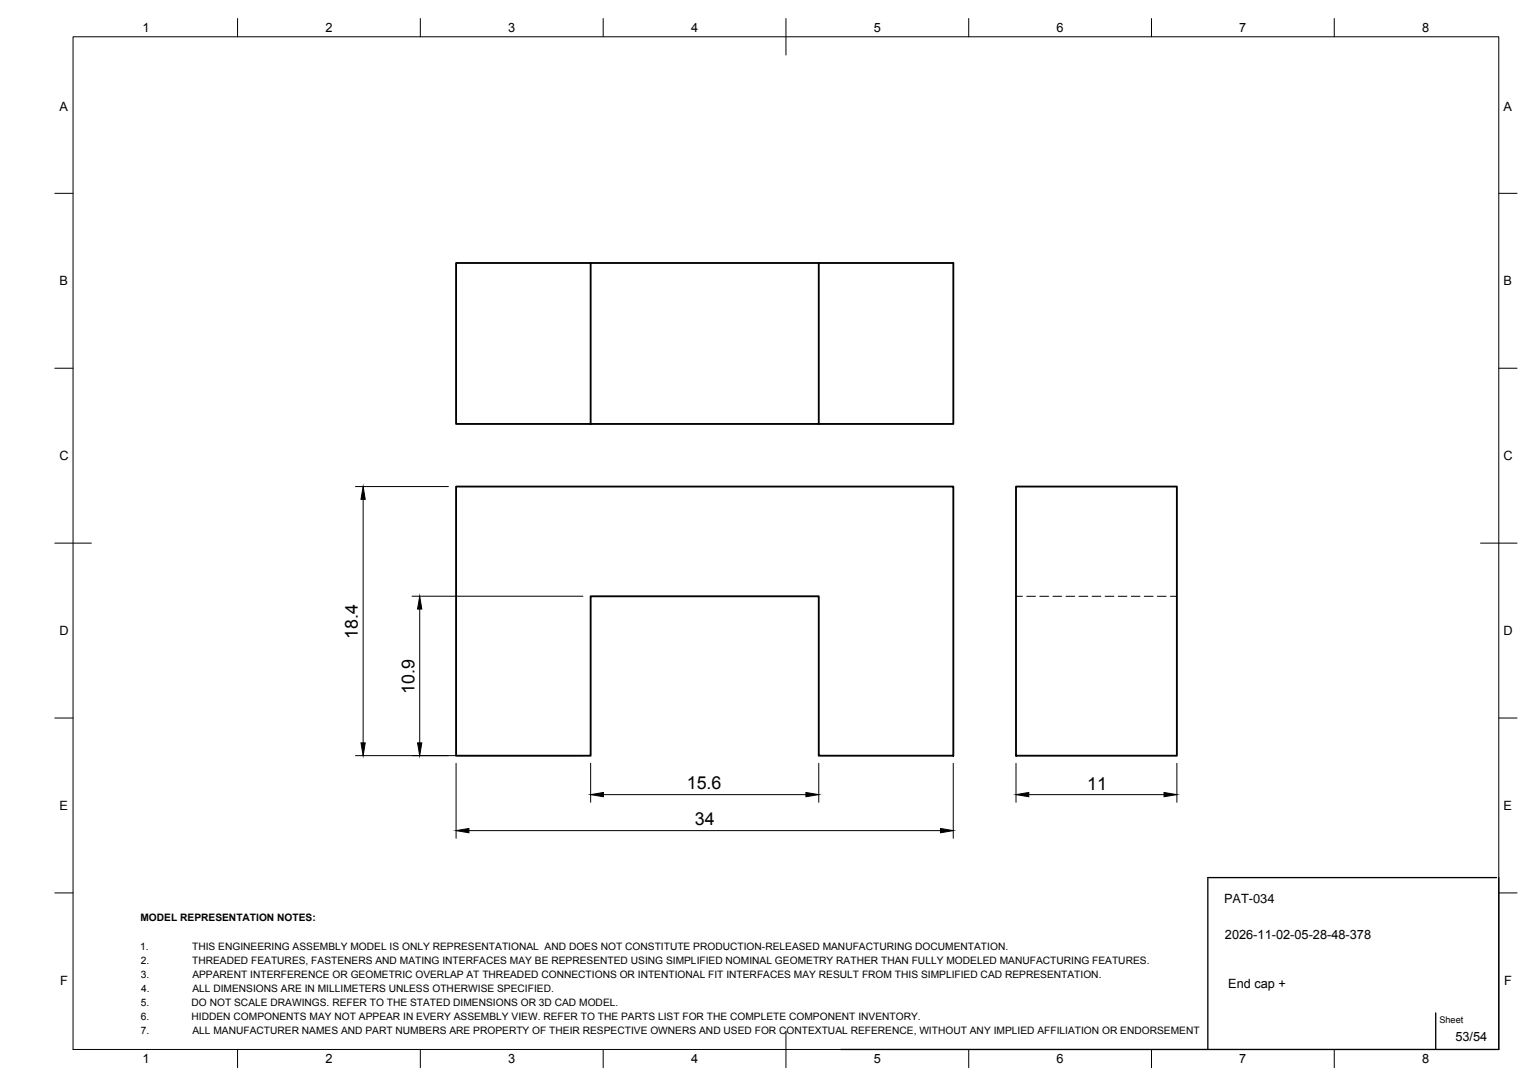
ISO-10303-21;
HEADER;
/* Generated by software containing ST-Developer
 * from STEP Tools, Inc. (www.steptools.com) 
 */

FILE_DESCRIPTION(
/* description */ ('Fatigue rig crank-slider'),
/* implementation_level */ '2;1');

FILE_NAME(
/* name */ 'End cap +.step',
/* time_stamp */ '2026-10-28T03:24:50-07:00',
/* author */ (''),
/* organization */ (''),
/* preprocessor_version */ 'ST-DEVELOPER v20.2',
/* originating_system */ 'Autodesk Translation Framework v15.17.0.0',
/* authorisation */ '');

FILE_SCHEMA (('AUTOMOTIVE_DESIGN { 1 0 10303 214 3 1 1 }'));
ENDSEC;

DATA;
#10=MECHANICAL_DESIGN_GEOMETRIC_PRESENTATION_REPRESENTATION('',(#640),#16911);
#531=SHAPE_REPRESENTATION_RELATIONSHIP('SRR','None',#17176,#581);
#581=ADVANCED_BREP_SHAPE_REPRESENTATION('',(#697),#16905);
#640=STYLED_ITEM('',(#17480),#697);
#697=MANIFOLD_SOLID_BREP('Body1',#8933);
#1162=PLANE('',#10382);
#1163=PLANE('',#10383);
#1164=PLANE('',#10384);
#1165=PLANE('',#10385);
#1166=PLANE('',#10386);
#1167=PLANE('',#10387);
#1168=PLANE('',#10388);
#1169=PLANE('',#10389);
#1170=PLANE('',#10390);
#1171=PLANE('',#10391);
#1666=FACE_OUTER_BOUND('',#2381,.T.);
#1667=FACE_OUTER_BOUND('',#2382,.T.);
#1668=FACE_OUTER_BOUND('',#2383,.T.);
#1669=FACE_OUTER_BOUND('',#2384,.T.);
#1670=FACE_OUTER_BOUND('',#2385,.T.);
#1671=FACE_OUTER_BOUND('',#2386,.T.);
#1672=FACE_OUTER_BOUND('',#2387,.T.);
#1673=FACE_OUTER_BOUND('',#2388,.T.);
#1674=FACE_OUTER_BOUND('',#2389,.T.);
#1675=FACE_OUTER_BOUND('',#2390,.T.);
#2381=EDGE_LOOP('',(#7900,#7901,#7902,#7903));
#2382=EDGE_LOOP('',(#7904,#7905,#7906,#7907));
#2383=EDGE_LOOP('',(#7908,#7909,#7910,#7911));
#2384=EDGE_LOOP('',(#7912,#7913,#7914,#7915));
#2385=EDGE_LOOP('',(#7916,#7917,#7918,#7919));
#2386=EDGE_LOOP('',(#7920,#7921,#7922,#7923));
#2387=EDGE_LOOP('',(#7924,#7925,#7926,#7927));
#2388=EDGE_LOOP('',(#7928,#7929,#7930,#7931));
#2389=EDGE_LOOP('',(#7932,#7933,#7934,#7935,#7936,#7937,#7938,#7939));
#2390=EDGE_LOOP('',(#7940,#7941,#7942,#7943,#7944,#7945,#7946,#7947));
#2985=LINE('',#16397,#3631);
#2986=LINE('',#16399,#3632);
#2987=LINE('',#16401,#3633);
#2988=LINE('',#16402,#3634);
#2989=LINE('',#16405,#3635);
#2990=LINE('',#16407,#3636);
#2991=LINE('',#16408,#3637);
#2992=LINE('',#16411,#3638);
#2993=LINE('',#16413,#3639);
#2994=LINE('',#16414,#3640);
#2995=LINE('',#16417,#3641);
#2996=LINE('',#16419,#3642);
#2997=LINE('',#16420,#3643);
#2998=LINE('',#16423,#3644);
#2999=LINE('',#16425,#3645);
#3000=LINE('',#16426,#3646);
#3001=LINE('',#16429,#3647);
#3002=LINE('',#16431,#3648);
#3003=LINE('',#16432,#3649);
#3004=LINE('',#16435,#3650);
#3005=LINE('',#16437,#3651);
#3006=LINE('',#16438,#3652);
#3007=LINE('',#16440,#3653);
#3008=LINE('',#16441,#3654);
#3631=VECTOR('',#12871,1.);
#3632=VECTOR('',#12872,1.);
#3633=VECTOR('',#12873,1.);
#3634=VECTOR('',#12874,1.);
#3635=VECTOR('',#12877,1.);
#3636=VECTOR('',#12878,1.);
#3637=VECTOR('',#12879,1.);
#3638=VECTOR('',#12882,1.);
#3639=VECTOR('',#12883,1.);
#3640=VECTOR('',#12884,1.);
#3641=VECTOR('',#12887,1.);
#3642=VECTOR('',#12888,1.);
#3643=VECTOR('',#12889,1.);
#3644=VECTOR('',#12892,1.);
#3645=VECTOR('',#12893,1.);
#3646=VECTOR('',#12894,1.);
#3647=VECTOR('',#12897,1.);
#3648=VECTOR('',#12898,1.);
#3649=VECTOR('',#12899,1.);
#3650=VECTOR('',#12902,1.);
#3651=VECTOR('',#12903,1.);
#3652=VECTOR('',#12904,1.);
#3653=VECTOR('',#12907,1.);
#3654=VECTOR('',#12908,1.);
#4801=VERTEX_POINT('',#16395);
#4802=VERTEX_POINT('',#16396);
#4803=VERTEX_POINT('',#16398);
#4804=VERTEX_POINT('',#16400);
#4805=VERTEX_POINT('',#16404);
#4806=VERTEX_POINT('',#16406);
#4807=VERTEX_POINT('',#16410);
#4808=VERTEX_POINT('',#16412);
#4809=VERTEX_POINT('',#16416);
#4810=VERTEX_POINT('',#16418);
#4811=VERTEX_POINT('',#16422);
#4812=VERTEX_POINT('',#16424);
#4813=VERTEX_POINT('',#16428);
#4814=VERTEX_POINT('',#16430);
#4815=VERTEX_POINT('',#16434);
#4816=VERTEX_POINT('',#16436);
#5848=EDGE_CURVE('',#4801,#4802,#2985,.T.);
#5849=EDGE_CURVE('',#4802,#4803,#2986,.T.);
#5850=EDGE_CURVE('',#4804,#4803,#2987,.T.);
#5851=EDGE_CURVE('',#4801,#4804,#2988,.T.);
#5852=EDGE_CURVE('',#4805,#4801,#2989,.T.);
#5853=EDGE_CURVE('',#4806,#4804,#2990,.T.);
#5854=EDGE_CURVE('',#4805,#4806,#2991,.T.);
#5855=EDGE_CURVE('',#4807,#4805,#2992,.T.);
#5856=EDGE_CURVE('',#4808,#4806,#2993,.T.);
#5857=EDGE_CURVE('',#4807,#4808,#2994,.T.);
#5858=EDGE_CURVE('',#4809,#4807,#2995,.T.);
#5859=EDGE_CURVE('',#4810,#4808,#2996,.T.);
#5860=EDGE_CURVE('',#4809,#4810,#2997,.T.);
#5861=EDGE_CURVE('',#4811,#4809,#2998,.T.);
#5862=EDGE_CURVE('',#4812,#4810,#2999,.T.);
#5863=EDGE_CURVE('',#4811,#4812,#3000,.T.);
#5864=EDGE_CURVE('',#4813,#4811,#3001,.T.);
#5865=EDGE_CURVE('',#4814,#4812,#3002,.T.);
#5866=EDGE_CURVE('',#4813,#4814,#3003,.T.);
#5867=EDGE_CURVE('',#4815,#4813,#3004,.T.);
#5868=EDGE_CURVE('',#4816,#4814,#3005,.T.);
#5869=EDGE_CURVE('',#4815,#4816,#3006,.T.);
#5870=EDGE_CURVE('',#4802,#4815,#3007,.T.);
#5871=EDGE_CURVE('',#4803,#4816,#3008,.T.);
#7900=ORIENTED_EDGE('',*,*,#5848,.T.);
#7901=ORIENTED_EDGE('',*,*,#5849,.T.);
#7902=ORIENTED_EDGE('',*,*,#5850,.F.);
#7903=ORIENTED_EDGE('',*,*,#5851,.F.);
#7904=ORIENTED_EDGE('',*,*,#5852,.T.);
#7905=ORIENTED_EDGE('',*,*,#5851,.T.);
#7906=ORIENTED_EDGE('',*,*,#5853,.F.);
#7907=ORIENTED_EDGE('',*,*,#5854,.F.);
#7908=ORIENTED_EDGE('',*,*,#5855,.T.);
#7909=ORIENTED_EDGE('',*,*,#5854,.T.);
#7910=ORIENTED_EDGE('',*,*,#5856,.F.);
#7911=ORIENTED_EDGE('',*,*,#5857,.F.);
#7912=ORIENTED_EDGE('',*,*,#5858,.T.);
#7913=ORIENTED_EDGE('',*,*,#5857,.T.);
#7914=ORIENTED_EDGE('',*,*,#5859,.F.);
#7915=ORIENTED_EDGE('',*,*,#5860,.F.);
#7916=ORIENTED_EDGE('',*,*,#5861,.T.);
#7917=ORIENTED_EDGE('',*,*,#5860,.T.);
#7918=ORIENTED_EDGE('',*,*,#5862,.F.);
#7919=ORIENTED_EDGE('',*,*,#5863,.F.);
#7920=ORIENTED_EDGE('',*,*,#5864,.T.);
#7921=ORIENTED_EDGE('',*,*,#5863,.T.);
#7922=ORIENTED_EDGE('',*,*,#5865,.F.);
#7923=ORIENTED_EDGE('',*,*,#5866,.F.);
#7924=ORIENTED_EDGE('',*,*,#5867,.T.);
#7925=ORIENTED_EDGE('',*,*,#5866,.T.);
#7926=ORIENTED_EDGE('',*,*,#5868,.F.);
#7927=ORIENTED_EDGE('',*,*,#5869,.F.);
#7928=ORIENTED_EDGE('',*,*,#5870,.T.);
#7929=ORIENTED_EDGE('',*,*,#5869,.T.);
#7930=ORIENTED_EDGE('',*,*,#5871,.F.);
#7931=ORIENTED_EDGE('',*,*,#5849,.F.);
#7932=ORIENTED_EDGE('',*,*,#5871,.T.);
#7933=ORIENTED_EDGE('',*,*,#5868,.T.);
#7934=ORIENTED_EDGE('',*,*,#5865,.T.);
#7935=ORIENTED_EDGE('',*,*,#5862,.T.);
#7936=ORIENTED_EDGE('',*,*,#5859,.T.);
#7937=ORIENTED_EDGE('',*,*,#5856,.T.);
#7938=ORIENTED_EDGE('',*,*,#5853,.T.);
#7939=ORIENTED_EDGE('',*,*,#5850,.T.);
#7940=ORIENTED_EDGE('',*,*,#5870,.F.);
#7941=ORIENTED_EDGE('',*,*,#5848,.F.);
#7942=ORIENTED_EDGE('',*,*,#5852,.F.);
#7943=ORIENTED_EDGE('',*,*,#5855,.F.);
#7944=ORIENTED_EDGE('',*,*,#5858,.F.);
#7945=ORIENTED_EDGE('',*,*,#5861,.F.);
#7946=ORIENTED_EDGE('',*,*,#5864,.F.);
#7947=ORIENTED_EDGE('',*,*,#5867,.F.);
#8804=ADVANCED_FACE('',(#1666),#1162,.T.);
#8805=ADVANCED_FACE('',(#1667),#1163,.T.);
#8806=ADVANCED_FACE('',(#1668),#1164,.T.);
#8807=ADVANCED_FACE('',(#1669),#1165,.T.);
#8808=ADVANCED_FACE('',(#1670),#1166,.T.);
#8809=ADVANCED_FACE('',(#1671),#1167,.T.);
#8810=ADVANCED_FACE('',(#1672),#1168,.T.);
#8811=ADVANCED_FACE('',(#1673),#1169,.T.);
#8812=ADVANCED_FACE('',(#1674),#1170,.T.);
#8813=ADVANCED_FACE('',(#1675),#1171,.F.);
#8933=CLOSED_SHELL('',(#8804,#8805,#8806,#8807,#8808,#8809,#8810,#8811,
#8812,#8813));
#10381=AXIS2_PLACEMENT_3D('',#16393,#12867,#12868);
#10382=AXIS2_PLACEMENT_3D('',#16394,#12869,#12870);
#10383=AXIS2_PLACEMENT_3D('',#16403,#12875,#12876);
#10384=AXIS2_PLACEMENT_3D('',#16409,#12880,#12881);
#10385=AXIS2_PLACEMENT_3D('',#16415,#12885,#12886);
#10386=AXIS2_PLACEMENT_3D('',#16421,#12890,#12891);
#10387=AXIS2_PLACEMENT_3D('',#16427,#12895,#12896);
#10388=AXIS2_PLACEMENT_3D('',#16433,#12900,#12901);
#10389=AXIS2_PLACEMENT_3D('',#16439,#12905,#12906);
#10390=AXIS2_PLACEMENT_3D('',#16442,#12909,#12910);
#10391=AXIS2_PLACEMENT_3D('',#16443,#12911,#12912);
#12867=DIRECTION('axis',(0.,0.,1.));
#12868=DIRECTION('refdir',(1.,0.,0.));
#12869=DIRECTION('center_axis',(0.,0.,1.));
#12870=DIRECTION('ref_axis',(0.,-1.,0.));
#12871=DIRECTION('',(0.,-1.,0.));
#12872=DIRECTION('',(1.,0.,0.));
#12873=DIRECTION('',(0.,-1.,0.));
#12874=DIRECTION('',(1.,0.,0.));
#12875=DIRECTION('center_axis',(0.,1.,0.));
#12876=DIRECTION('ref_axis',(0.,0.,1.));
#12877=DIRECTION('',(0.,0.,1.));
#12878=DIRECTION('',(0.,0.,1.));
#12879=DIRECTION('',(1.,0.,0.));
#12880=DIRECTION('center_axis',(0.,0.,-1.));
#12881=DIRECTION('ref_axis',(0.,1.,0.));
#12882=DIRECTION('',(0.,1.,0.));
#12883=DIRECTION('',(0.,1.,0.));
#12884=DIRECTION('',(1.,0.,0.));
#12885=DIRECTION('center_axis',(0.,-1.,0.));
#12886=DIRECTION('ref_axis',(0.,0.,-1.));
#12887=DIRECTION('',(0.,0.,-1.));
#12888=DIRECTION('',(0.,0.,-1.));
#12889=DIRECTION('',(1.,0.,0.));
#12890=DIRECTION('center_axis',(0.,0.,-1.));
#12891=DIRECTION('ref_axis',(0.,1.,0.));
#12892=DIRECTION('',(0.,1.,0.));
#12893=DIRECTION('',(0.,1.,0.));
#12894=DIRECTION('',(1.,0.,0.));
#12895=DIRECTION('center_axis',(0.,1.,0.));
#12896=DIRECTION('ref_axis',(0.,0.,1.));
#12897=DIRECTION('',(0.,0.,1.));
#12898=DIRECTION('',(0.,0.,1.));
#12899=DIRECTION('',(1.,0.,0.));
#12900=DIRECTION('center_axis',(0.,0.,-1.));
#12901=DIRECTION('ref_axis',(0.,1.,0.));
#12902=DIRECTION('',(0.,1.,0.));
#12903=DIRECTION('',(0.,1.,0.));
#12904=DIRECTION('',(1.,0.,0.));
#12905=DIRECTION('center_axis',(0.,-1.,0.));
#12906=DIRECTION('ref_axis',(0.,0.,-1.));
#12907=DIRECTION('',(0.,0.,-1.));
#12908=DIRECTION('',(0.,0.,-1.));
#12909=DIRECTION('center_axis',(1.,0.,0.));
#12910=DIRECTION('ref_axis',(0.,0.,-1.));
#12911=DIRECTION('center_axis',(1.,0.,0.));
#12912=DIRECTION('ref_axis',(0.,0.,-1.));
#16393=CARTESIAN_POINT('',(0.,0.,0.));
#16394=CARTESIAN_POINT('Origin',(1.97,1.7,2.3));
#16395=CARTESIAN_POINT('',(1.97,1.7,2.3));
#16396=CARTESIAN_POINT('',(1.97,-1.7,2.3));
#16397=CARTESIAN_POINT('',(1.97,1.7,2.3));
#16398=CARTESIAN_POINT('',(3.07,-1.7,2.3));
#16399=CARTESIAN_POINT('',(1.97,-1.7,2.3));
#16400=CARTESIAN_POINT('',(3.07,1.7,2.3));
#16401=CARTESIAN_POINT('',(3.07,1.7,2.3));
#16402=CARTESIAN_POINT('',(1.97,1.7,2.3));
#16403=CARTESIAN_POINT('Origin',(1.97,1.7,0.46));
#16404=CARTESIAN_POINT('',(1.97,1.7,0.46));
#16405=CARTESIAN_POINT('',(1.97,1.7,0.46));
#16406=CARTESIAN_POINT('',(3.07,1.7,0.46));
#16407=CARTESIAN_POINT('',(3.07,1.7,0.46));
#16408=CARTESIAN_POINT('',(1.97,1.7,0.46));
#16409=CARTESIAN_POINT('Origin',(1.97,0.78,0.46));
#16410=CARTESIAN_POINT('',(1.97,0.78,0.46));
#16411=CARTESIAN_POINT('',(1.97,0.78,0.46));
#16412=CARTESIAN_POINT('',(3.07,0.78,0.46));
#16413=CARTESIAN_POINT('',(3.07,0.78,0.46));
#16414=CARTESIAN_POINT('',(1.97,0.78,0.46));
#16415=CARTESIAN_POINT('Origin',(1.97,0.78,1.55));
#16416=CARTESIAN_POINT('',(1.97,0.78,1.55));
#16417=CARTESIAN_POINT('',(1.97,0.78,1.55));
#16418=CARTESIAN_POINT('',(3.07,0.78,1.55));
#16419=CARTESIAN_POINT('',(3.07,0.78,1.55));
#16420=CARTESIAN_POINT('',(1.97,0.78,1.55));
#16421=CARTESIAN_POINT('Origin',(1.97,-0.78,1.55));
#16422=CARTESIAN_POINT('',(1.97,-0.78,1.55));
#16423=CARTESIAN_POINT('',(1.97,-0.78,1.55));
#16424=CARTESIAN_POINT('',(3.07,-0.78,1.55));
#16425=CARTESIAN_POINT('',(3.07,-0.78,1.55));
#16426=CARTESIAN_POINT('',(1.97,-0.78,1.55));
#16427=CARTESIAN_POINT('Origin',(1.97,-0.78,0.46));
#16428=CARTESIAN_POINT('',(1.97,-0.78,0.46));
#16429=CARTESIAN_POINT('',(1.97,-0.78,0.46));
#16430=CARTESIAN_POINT('',(3.07,-0.78,0.46));
#16431=CARTESIAN_POINT('',(3.07,-0.78,0.46));
#16432=CARTESIAN_POINT('',(1.97,-0.78,0.46));
#16433=CARTESIAN_POINT('Origin',(1.97,-1.7,0.46));
#16434=CARTESIAN_POINT('',(1.97,-1.7,0.46));
#16435=CARTESIAN_POINT('',(1.97,-1.7,0.46));
#16436=CARTESIAN_POINT('',(3.07,-1.7,0.46));
#16437=CARTESIAN_POINT('',(3.07,-1.7,0.46));
#16438=CARTESIAN_POINT('',(1.97,-1.7,0.46));
#16439=CARTESIAN_POINT('Origin',(1.97,-1.7,2.3));
#16440=CARTESIAN_POINT('',(1.97,-1.7,2.3));
#16441=CARTESIAN_POINT('',(3.07,-1.7,2.3));
#16442=CARTESIAN_POINT('Origin',(3.07,0.,1.38));
#16443=CARTESIAN_POINT('Origin',(1.97,0.,1.38));
#16846=UNCERTAINTY_MEASURE_WITH_UNIT(LENGTH_MEASURE(0.001),#16912,
'DISTANCE_ACCURACY_VALUE',
'Maximum model space distance between geometric entities at asserted c
onnectivities');
#16852=UNCERTAINTY_MEASURE_WITH_UNIT(LENGTH_MEASURE(0.001),#16912,
'DISTANCE_ACCURACY_VALUE',
'Maximum model space distance between geometric entities at asserted c
onnectivities');
#16905=(
GEOMETRIC_REPRESENTATION_CONTEXT(3)
GLOBAL_UNCERTAINTY_ASSIGNED_CONTEXT((#16846))
GLOBAL_UNIT_ASSIGNED_CONTEXT((#16912,#16914,#16915))
REPRESENTATION_CONTEXT('','3D')
);
#16911=(
GEOMETRIC_REPRESENTATION_CONTEXT(3)
GLOBAL_UNCERTAINTY_ASSIGNED_CONTEXT((#16852))
GLOBAL_UNIT_ASSIGNED_CONTEXT((#16912,#16914,#16915))
REPRESENTATION_CONTEXT('','3D')
);
#16912=(
LENGTH_UNIT()
NAMED_UNIT(*)
SI_UNIT(.CENTI.,.METRE.)
);
#16914=(
NAMED_UNIT(*)
PLANE_ANGLE_UNIT()
SI_UNIT($,.RADIAN.)
);
#16915=(
NAMED_UNIT(*)
SI_UNIT($,.STERADIAN.)
SOLID_ANGLE_UNIT()
);
#16968=SHAPE_DEFINITION_REPRESENTATION(#17040,#17176);
#17040=PRODUCT_DEFINITION_SHAPE('',$,#17235);
#17176=SHAPE_REPRESENTATION('',(#10381),#16905);
#17182=PRODUCT_DEFINITION_CONTEXT('part definition',#17358,'design');
#17235=PRODUCT_DEFINITION('End cap +','End cap +',#17293,#17182);
#17293=PRODUCT_DEFINITION_FORMATION('',$,#17412);
#17358=APPLICATION_CONTEXT(
'Core Data for Automotive Mechanical Design Process');
#17359=PRODUCT_CONTEXT('part definition',#17358,'mechanical');
#17412=PRODUCT('End cap +','End cap +','End cap +',(#17359));
#17474=COLOUR_RGB('Sky Blue',0.24,0.69,0.87);
#17475=FILL_AREA_STYLE_COLOUR('',#17474);
#17476=FILL_AREA_STYLE('',(#17475));
#17477=SURFACE_STYLE_FILL_AREA(#17476);
#17478=SURFACE_SIDE_STYLE('',(#17477));
#17479=SURFACE_STYLE_USAGE(.BOTH.,#17478);
#17480=PRESENTATION_STYLE_ASSIGNMENT((#17479));
ENDSEC;
END-ISO-10303-21;
